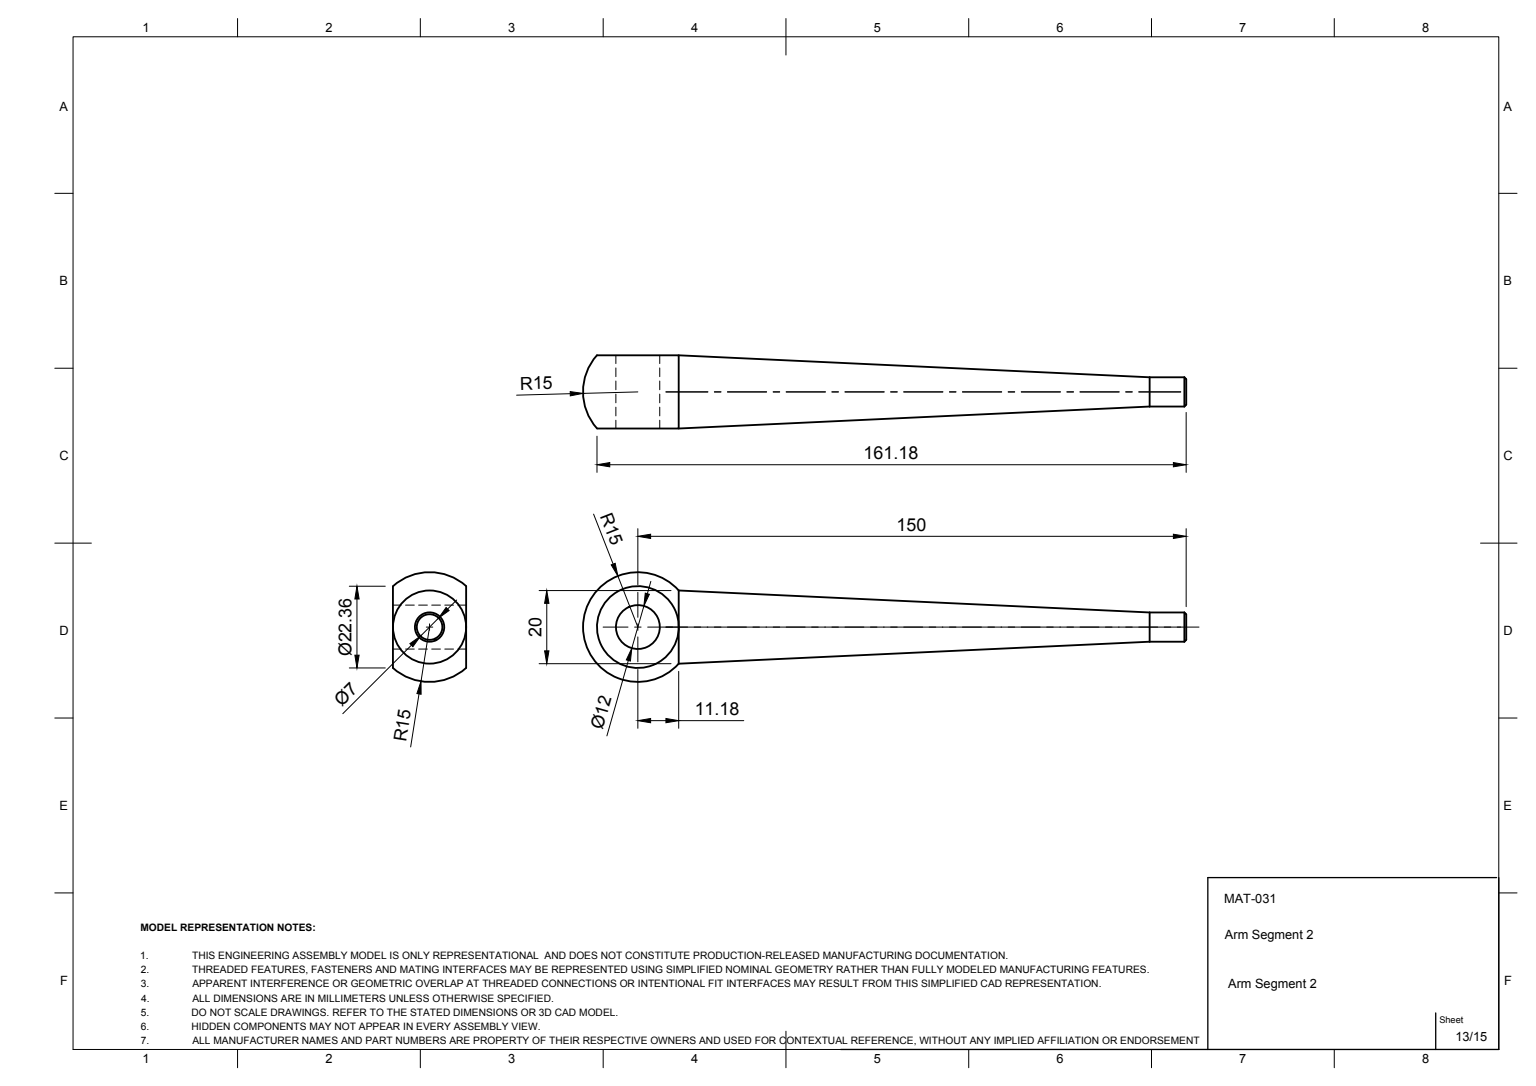
ISO-10303-21;
HEADER;
/* Generated by software containing ST-Developer
 * from STEP Tools, Inc. (www.steptools.com) 
 */

FILE_DESCRIPTION(
/* description */ ('STEP AP214'),
/* implementation_level */ '2;1');

FILE_NAME(
/* name */ 'Arm Segment 2.step',
/* time_stamp */ '2026-11-14T06:58:01-08:00',
/* author */ (''),
/* organization */ (''),
/* preprocessor_version */ 'ST-DEVELOPER v20.2',
/* originating_system */ 'Autodesk Translation Framework v15.17.0.0',
/* authorisation */ '');

FILE_SCHEMA (('AUTOMOTIVE_DESIGN { 1 0 10303 214 3 1 1 }'));
ENDSEC;

DATA;
#10=MECHANICAL_DESIGN_GEOMETRIC_PRESENTATION_REPRESENTATION('',(#1156),#38635);
#91=SPHERICAL_SURFACE('',#18197,15.);
#92=SPHERICAL_SURFACE('',#18205,15.);
#879=FACE_BOUND('',#2902,.T.);
#880=FACE_BOUND('',#2904,.T.);
#1031=CONICAL_SURFACE('',#18209,4.,0.0465431041182806);
#1032=CONICAL_SURFACE('',#18213,3.5,0.785398163397448);
#1122=SHAPE_REPRESENTATION_RELATIONSHIP('SRR','None',#38695,#1136);
#1136=ADVANCED_BREP_SHAPE_REPRESENTATION('',(#1182),#38631);
#1156=STYLED_ITEM('',(#38765),#1182);
#1182=MANIFOLD_SOLID_BREP('Body1',#17622);
#1268=PLANE('',#18215);
#1269=PLANE('',#18216);
#1270=PLANE('',#18217);
#1871=FACE_OUTER_BOUND('',#2894,.T.);
#1872=FACE_OUTER_BOUND('',#2895,.T.);
#1873=FACE_OUTER_BOUND('',#2896,.T.);
#1874=FACE_OUTER_BOUND('',#2897,.T.);
#1875=FACE_OUTER_BOUND('',#2898,.T.);
#1876=FACE_OUTER_BOUND('',#2899,.T.);
#1877=FACE_OUTER_BOUND('',#2900,.T.);
#1878=FACE_OUTER_BOUND('',#2901,.T.);
#1879=FACE_OUTER_BOUND('',#2903,.T.);
#2894=EDGE_LOOP('',(#11997,#11998,#11999,#12000));
#2895=EDGE_LOOP('',(#12001,#12002,#12003,#12004));
#2896=EDGE_LOOP('',(#12005,#12006,#12007,#12008));
#2897=EDGE_LOOP('',(#12009,#12010,#12011,#12012,#12013));
#2898=EDGE_LOOP('',(#12014,#12015,#12016,#12017));
#2899=EDGE_LOOP('',(#12018,#12019,#12020,#12021));
#2900=EDGE_LOOP('',(#12022));
#2901=EDGE_LOOP('',(#12023,#12024));
#2902=EDGE_LOOP('',(#12025));
#2903=EDGE_LOOP('',(#12026,#12027));
#2904=EDGE_LOOP('',(#12028));
#3908=LINE('',#32988,#4852);
#3909=LINE('',#32996,#4853);
#3910=LINE('',#33000,#4854);
#3911=LINE('',#33004,#4855);
#4852=VECTOR('',#20787,6.);
#4853=VECTOR('',#20800,4.);
#4854=VECTOR('',#20805,4.);
#4855=VECTOR('',#20810,3.5);
#5769=CIRCLE('',#18198,15.);
#5770=CIRCLE('',#18199,11.1803398874989);
#5771=CIRCLE('',#18200,10.);
#5772=CIRCLE('',#18201,11.1803398874989);
#5773=CIRCLE('',#18203,6.);
#5774=CIRCLE('',#18204,6.);
#5775=CIRCLE('',#18206,11.1803398874989);
#5776=CIRCLE('',#18207,10.);
#5777=CIRCLE('',#18208,11.1803398874989);
#5778=CIRCLE('',#18210,4.);
#5779=CIRCLE('',#18212,4.);
#5780=CIRCLE('',#18214,3.5);
#6863=VERTEX_POINT('',#32976);
#6864=VERTEX_POINT('',#32977);
#6865=VERTEX_POINT('',#32979);
#6866=VERTEX_POINT('',#32981);
#6867=VERTEX_POINT('',#32985);
#6868=VERTEX_POINT('',#32987);
#6869=VERTEX_POINT('',#32995);
#6870=VERTEX_POINT('',#32999);
#6871=VERTEX_POINT('',#33003);
#8785=EDGE_CURVE('',#6863,#6864,#5769,.T.);
#8786=EDGE_CURVE('',#6863,#6865,#5770,.T.);
#8787=EDGE_CURVE('',#6865,#6866,#5771,.T.);
#8788=EDGE_CURVE('',#6866,#6864,#5772,.T.);
#8789=EDGE_CURVE('',#6867,#6867,#5773,.T.);
#8790=EDGE_CURVE('',#6867,#6868,#3908,.T.);
#8791=EDGE_CURVE('',#6868,#6868,#5774,.T.);
#8792=EDGE_CURVE('',#6864,#6866,#5775,.T.);
#8793=EDGE_CURVE('',#6866,#6865,#5776,.T.);
#8794=EDGE_CURVE('',#6865,#6863,#5777,.T.);
#8795=EDGE_CURVE('',#6865,#6869,#3909,.T.);
#8796=EDGE_CURVE('',#6869,#6869,#5778,.T.);
#8797=EDGE_CURVE('',#6869,#6870,#3910,.T.);
#8798=EDGE_CURVE('',#6870,#6870,#5779,.T.);
#8799=EDGE_CURVE('',#6870,#6871,#3911,.T.);
#8800=EDGE_CURVE('',#6871,#6871,#5780,.T.);
#11997=ORIENTED_EDGE('',*,*,#8785,.F.);
#11998=ORIENTED_EDGE('',*,*,#8786,.T.);
#11999=ORIENTED_EDGE('',*,*,#8787,.T.);
#12000=ORIENTED_EDGE('',*,*,#8788,.T.);
#12001=ORIENTED_EDGE('',*,*,#8789,.F.);
#12002=ORIENTED_EDGE('',*,*,#8790,.T.);
#12003=ORIENTED_EDGE('',*,*,#8791,.T.);
#12004=ORIENTED_EDGE('',*,*,#8790,.F.);
#12005=ORIENTED_EDGE('',*,*,#8785,.T.);
#12006=ORIENTED_EDGE('',*,*,#8792,.T.);
#12007=ORIENTED_EDGE('',*,*,#8793,.T.);
#12008=ORIENTED_EDGE('',*,*,#8794,.T.);
#12009=ORIENTED_EDGE('',*,*,#8787,.F.);
#12010=ORIENTED_EDGE('',*,*,#8795,.T.);
#12011=ORIENTED_EDGE('',*,*,#8796,.T.);
#12012=ORIENTED_EDGE('',*,*,#8795,.F.);
#12013=ORIENTED_EDGE('',*,*,#8793,.F.);
#12014=ORIENTED_EDGE('',*,*,#8796,.F.);
#12015=ORIENTED_EDGE('',*,*,#8797,.T.);
#12016=ORIENTED_EDGE('',*,*,#8798,.T.);
#12017=ORIENTED_EDGE('',*,*,#8797,.F.);
#12018=ORIENTED_EDGE('',*,*,#8798,.F.);
#12019=ORIENTED_EDGE('',*,*,#8799,.T.);
#12020=ORIENTED_EDGE('',*,*,#8800,.T.);
#12021=ORIENTED_EDGE('',*,*,#8799,.F.);
#12022=ORIENTED_EDGE('',*,*,#8800,.F.);
#12023=ORIENTED_EDGE('',*,*,#8788,.F.);
#12024=ORIENTED_EDGE('',*,*,#8792,.F.);
#12025=ORIENTED_EDGE('',*,*,#8791,.F.);
#12026=ORIENTED_EDGE('',*,*,#8794,.F.);
#12027=ORIENTED_EDGE('',*,*,#8786,.F.);
#12028=ORIENTED_EDGE('',*,*,#8789,.T.);
#16343=CYLINDRICAL_SURFACE('',#18202,6.);
#16344=CYLINDRICAL_SURFACE('',#18211,4.);
#16830=ADVANCED_FACE('',(#1871),#91,.T.);
#16831=ADVANCED_FACE('',(#1872),#16343,.F.);
#16832=ADVANCED_FACE('',(#1873),#92,.T.);
#16833=ADVANCED_FACE('',(#1874),#1031,.T.);
#16834=ADVANCED_FACE('',(#1875),#16344,.T.);
#16835=ADVANCED_FACE('',(#1876),#1032,.T.);
#16836=ADVANCED_FACE('',(#1877),#1268,.F.);
#16837=ADVANCED_FACE('',(#1878,#879),#1269,.F.);
#16838=ADVANCED_FACE('',(#1879,#880),#1270,.F.);
#17622=CLOSED_SHELL('',(#16830,#16831,#16832,#16833,#16834,#16835,#16836,
#16837,#16838));
#18196=AXIS2_PLACEMENT_3D('',#32974,#20771,#20772);
#18197=AXIS2_PLACEMENT_3D('',#32975,#20773,#20774);
#18198=AXIS2_PLACEMENT_3D('',#32978,#20775,#20776);
#18199=AXIS2_PLACEMENT_3D('',#32980,#20777,#20778);
#18200=AXIS2_PLACEMENT_3D('',#32982,#20779,#20780);
#18201=AXIS2_PLACEMENT_3D('',#32983,#20781,#20782);
#18202=AXIS2_PLACEMENT_3D('',#32984,#20783,#20784);
#18203=AXIS2_PLACEMENT_3D('',#32986,#20785,#20786);
#18204=AXIS2_PLACEMENT_3D('',#32989,#20788,#20789);
#18205=AXIS2_PLACEMENT_3D('',#32990,#20790,#20791);
#18206=AXIS2_PLACEMENT_3D('',#32991,#20792,#20793);
#18207=AXIS2_PLACEMENT_3D('',#32992,#20794,#20795);
#18208=AXIS2_PLACEMENT_3D('',#32993,#20796,#20797);
#18209=AXIS2_PLACEMENT_3D('',#32994,#20798,#20799);
#18210=AXIS2_PLACEMENT_3D('',#32997,#20801,#20802);
#18211=AXIS2_PLACEMENT_3D('',#32998,#20803,#20804);
#18212=AXIS2_PLACEMENT_3D('',#33001,#20806,#20807);
#18213=AXIS2_PLACEMENT_3D('',#33002,#20808,#20809);
#18214=AXIS2_PLACEMENT_3D('',#33005,#20811,#20812);
#18215=AXIS2_PLACEMENT_3D('',#33006,#20813,#20814);
#18216=AXIS2_PLACEMENT_3D('',#33007,#20815,#20816);
#18217=AXIS2_PLACEMENT_3D('',#33008,#20817,#20818);
#20771=DIRECTION('axis',(0.,0.,1.));
#20772=DIRECTION('refdir',(1.,0.,0.));
#20773=DIRECTION('center_axis',(0.,6.12323399573677E-17,-1.));
#20774=DIRECTION('ref_axis',(0.,1.,0.));
#20775=DIRECTION('center_axis',(-1.,1.22464679914735E-16,0.));
#20776=DIRECTION('ref_axis',(-1.22464679914735E-16,-1.,0.));
#20777=DIRECTION('center_axis',(0.,0.,1.));
#20778=DIRECTION('ref_axis',(1.,0.,0.));
#20779=DIRECTION('center_axis',(-1.,0.,0.));
#20780=DIRECTION('ref_axis',(0.,0.,1.));
#20781=DIRECTION('center_axis',(0.,0.,-1.));
#20782=DIRECTION('ref_axis',(-1.,0.,0.));
#20783=DIRECTION('center_axis',(0.,0.,1.));
#20784=DIRECTION('ref_axis',(1.,0.,0.));
#20785=DIRECTION('center_axis',(0.,0.,1.));
#20786=DIRECTION('ref_axis',(1.,0.,0.));
#20787=DIRECTION('',(0.,0.,1.));
#20788=DIRECTION('center_axis',(0.,0.,1.));
#20789=DIRECTION('ref_axis',(1.,0.,0.));
#20790=DIRECTION('center_axis',(0.,6.12323399573677E-17,-1.));
#20791=DIRECTION('ref_axis',(0.,1.,0.));
#20792=DIRECTION('center_axis',(0.,0.,-1.));
#20793=DIRECTION('ref_axis',(-1.,0.,0.));
#20794=DIRECTION('center_axis',(-1.,0.,0.));
#20795=DIRECTION('ref_axis',(0.,0.,1.));
#20796=DIRECTION('center_axis',(0.,0.,1.));
#20797=DIRECTION('ref_axis',(1.,0.,0.));
#20798=DIRECTION('center_axis',(-1.,0.,0.));
#20799=DIRECTION('ref_axis',(0.,0.,1.));
#20800=DIRECTION('',(0.99891706524393,5.69782866448938E-18,0.0465263018566368));
#20801=DIRECTION('center_axis',(-1.,0.,0.));
#20802=DIRECTION('ref_axis',(0.,0.,1.));
#20803=DIRECTION('center_axis',(-1.,0.,0.));
#20804=DIRECTION('ref_axis',(0.,0.,1.));
#20805=DIRECTION('',(1.,0.,0.));
#20806=DIRECTION('center_axis',(-1.,0.,0.));
#20807=DIRECTION('ref_axis',(0.,0.,1.));
#20808=DIRECTION('center_axis',(-1.,0.,0.));
#20809=DIRECTION('ref_axis',(0.,0.,1.));
#20810=DIRECTION('',(0.707106781186548,8.65956056235493E-17,0.707106781186547));
#20811=DIRECTION('center_axis',(-1.,0.,0.));
#20812=DIRECTION('ref_axis',(0.,0.,1.));
#20813=DIRECTION('center_axis',(-1.,0.,0.));
#20814=DIRECTION('ref_axis',(0.,0.,1.));
#20815=DIRECTION('center_axis',(0.,0.,-1.));
#20816=DIRECTION('ref_axis',(-1.,0.,0.));
#20817=DIRECTION('center_axis',(0.,0.,1.));
#20818=DIRECTION('ref_axis',(1.,0.,0.));
#32974=CARTESIAN_POINT('',(0.,0.,0.));
#32975=CARTESIAN_POINT('Origin',(0.,0.,0.));
#32976=CARTESIAN_POINT('',(-1.36919674566051E-15,-11.1803398874989,-10.));
#32977=CARTESIAN_POINT('',(-1.36919674566051E-15,-11.1803398874989,10.));
#32978=CARTESIAN_POINT('Origin',(0.,0.,0.));
#32979=CARTESIAN_POINT('',(11.1803398874989,0.,-10.));
#32980=CARTESIAN_POINT('Origin',(0.,0.,-10.));
#32981=CARTESIAN_POINT('',(11.1803398874989,0.,10.));
#32982=CARTESIAN_POINT('Origin',(11.1803398874989,0.,0.));
#32983=CARTESIAN_POINT('Origin',(0.,0.,10.));
#32984=CARTESIAN_POINT('Origin',(0.,0.,-10.));
#32985=CARTESIAN_POINT('',(-6.,-7.34788079488412E-16,-10.));
#32986=CARTESIAN_POINT('Origin',(0.,0.,-10.));
#32987=CARTESIAN_POINT('',(-6.,-7.34788079488412E-16,10.));
#32988=CARTESIAN_POINT('',(-6.,-7.34788079488412E-16,-10.));
#32989=CARTESIAN_POINT('Origin',(0.,0.,10.));
#32990=CARTESIAN_POINT('Origin',(0.,0.,0.));
#32991=CARTESIAN_POINT('Origin',(0.,0.,10.));
#32992=CARTESIAN_POINT('Origin',(11.1803398874989,0.,0.));
#32993=CARTESIAN_POINT('Origin',(0.,0.,-10.));
#32994=CARTESIAN_POINT('Origin',(140.,0.,0.));
#32995=CARTESIAN_POINT('',(140.,-4.89858719658941E-16,-4.));
#32996=CARTESIAN_POINT('',(140.,-4.89858719658941E-16,-4.));
#32997=CARTESIAN_POINT('Origin',(140.,0.,0.));
#32998=CARTESIAN_POINT('Origin',(-71.1905382258649,0.,0.));
#32999=CARTESIAN_POINT('',(149.5,-4.89858719658941E-16,-4.));
#33000=CARTESIAN_POINT('',(-71.1905382258649,-4.89858719658941E-16,-4.));
#33001=CARTESIAN_POINT('Origin',(149.5,0.,0.));
#33002=CARTESIAN_POINT('Origin',(150.,0.,0.));
#33003=CARTESIAN_POINT('',(150.,-4.28626379701574E-16,-3.5));
#33004=CARTESIAN_POINT('',(150.,-4.28626379701574E-16,-3.5));
#33005=CARTESIAN_POINT('Origin',(150.,0.,0.));
#33006=CARTESIAN_POINT('Origin',(150.,0.,0.));
#33007=CARTESIAN_POINT('Origin',(11.1803398874989,-15.,10.));
#33008=CARTESIAN_POINT('Origin',(11.1803398874989,-15.,-10.));
#38615=UNCERTAINTY_MEASURE_WITH_UNIT(LENGTH_MEASURE(0.01),#38636,
'DISTANCE_ACCURACY_VALUE',
'Maximum model space distance between geometric entities at asserted c
onnectivities');
#38619=UNCERTAINTY_MEASURE_WITH_UNIT(LENGTH_MEASURE(0.01),#38636,
'DISTANCE_ACCURACY_VALUE',
'Maximum model space distance between geometric entities at asserted c
onnectivities');
#38631=(
GEOMETRIC_REPRESENTATION_CONTEXT(3)
GLOBAL_UNCERTAINTY_ASSIGNED_CONTEXT((#38615))
GLOBAL_UNIT_ASSIGNED_CONTEXT((#38636,#38638,#38639))
REPRESENTATION_CONTEXT('','3D')
);
#38635=(
GEOMETRIC_REPRESENTATION_CONTEXT(3)
GLOBAL_UNCERTAINTY_ASSIGNED_CONTEXT((#38619))
GLOBAL_UNIT_ASSIGNED_CONTEXT((#38636,#38638,#38639))
REPRESENTATION_CONTEXT('','3D')
);
#38636=(
LENGTH_UNIT()
NAMED_UNIT(*)
SI_UNIT(.MILLI.,.METRE.)
);
#38638=(
NAMED_UNIT(*)
PLANE_ANGLE_UNIT()
SI_UNIT($,.RADIAN.)
);
#38639=(
NAMED_UNIT(*)
SI_UNIT($,.STERADIAN.)
SOLID_ANGLE_UNIT()
);
#38651=SHAPE_DEFINITION_REPRESENTATION(#38666,#38695);
#38666=PRODUCT_DEFINITION_SHAPE('',$,#38711);
#38695=SHAPE_REPRESENTATION('',(#18196),#38631);
#38699=PRODUCT_DEFINITION_CONTEXT('part definition',#38746,'design');
#38711=PRODUCT_DEFINITION('Arm Segment 2','Arm Segment 2',#38726,#38699);
#38726=PRODUCT_DEFINITION_FORMATION('',$,#38759);
#38746=APPLICATION_CONTEXT(
'Core Data for Automotive Mechanical Design Process');
#38747=PRODUCT_CONTEXT('part definition',#38746,'mechanical');
#38759=PRODUCT('Arm Segment 2','Arm Segment 2',$,(#38747));
#38765=PRESENTATION_STYLE_ASSIGNMENT((#38772));
#38772=SURFACE_STYLE_USAGE(.BOTH.,#38779);
#38779=SURFACE_SIDE_STYLE('',(#38786));
#38786=SURFACE_STYLE_FILL_AREA(#38793);
#38793=FILL_AREA_STYLE('Opaque(227,224,212)',(#38800));
#38800=FILL_AREA_STYLE_COLOUR('Opaque(227,224,212)',#38807);
#38807=COLOUR_RGB('Opaque(227,224,212)',0.890196078431372,0.87843137254902,
0.831372549019608);
ENDSEC;
END-ISO-10303-21;
